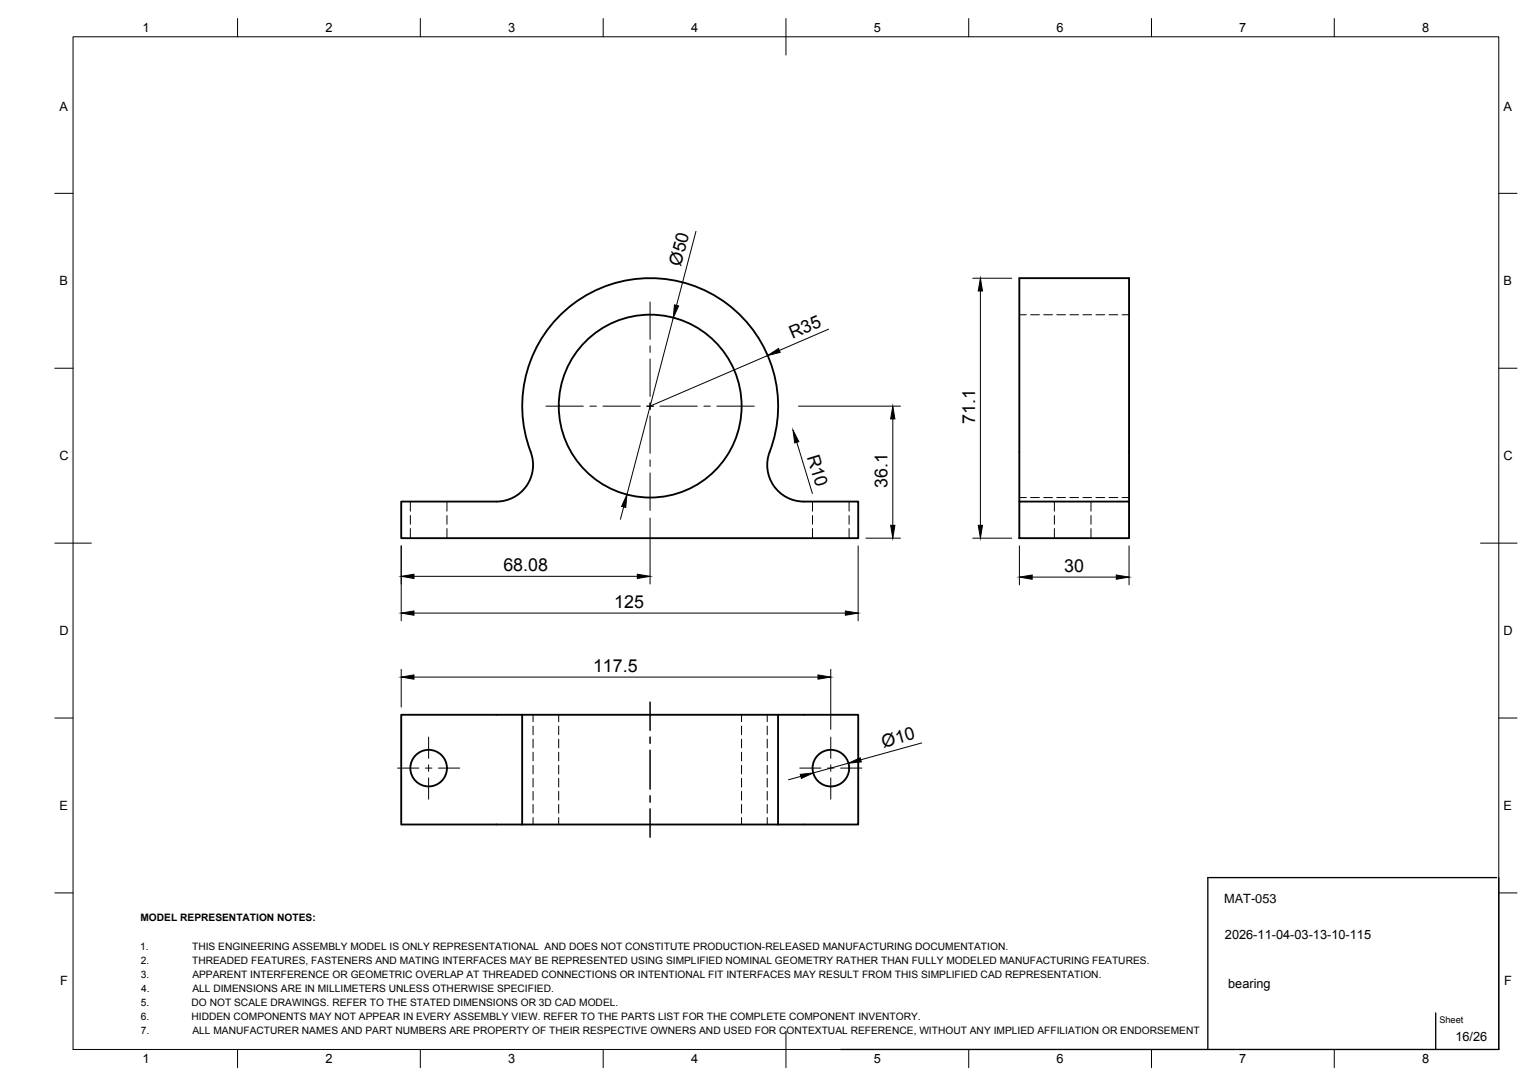
ISO-10303-21;
HEADER;
FILE_DESCRIPTION (('STEP AP214'),
    '1' );
FILE_NAME ('bearing.step',
    '2026-10-10T03:43:58',
    ( '' ),
    ( '' ),
    'SwSTEP 2.0',
    'SolidWorks 2026',
    '' );
FILE_SCHEMA (( 'AUTOMOTIVE_DESIGN' ));
ENDSEC;

DATA;
#80=( NAMED_UNIT ( * ) PLANE_ANGLE_UNIT ( ) SI_UNIT ( $, .RADIAN. ) );
#94=EDGE_CURVE ( 'NONE', #10885, #49715, #23914, .T. ) ;
#206=EDGE_CURVE ( 'NONE', #68800, #69210, #4699, .T. ) ;
#264=( NAMED_UNIT ( * ) SI_UNIT ( $, .STERADIAN. ) SOLID_ANGLE_UNIT ( ) );
#321=EDGE_CURVE ( 'NONE', #69231, #19186, #17084, .T. ) ;
#468=DIRECTION ( 'NONE',  ( -0.000000000000000000, -0.000000000000000000, -1.000000000000000000 ) ) ;
#638=ORIENTED_EDGE ( 'NONE', *, *, #35254, .T. ) ;
#689=ORIENTED_EDGE ( 'NONE', *, *, #206, .F. ) ;
#727=DIRECTION ( 'NONE',  ( -0.000000000000000000, -0.000000000000000000, -1.000000000000000000 ) ) ;
#740=CARTESIAN_POINT ( 'NONE',  ( -56.92000000000000171, -36.09918303830819752, 30.00000000000000000 ) ) ;
#794=LINE ( 'NONE', #10991, #2437 ) ;
#842=ORIENTED_EDGE ( 'NONE', *, *, #61547, .F. ) ;
#853=ORIENTED_EDGE ( 'NONE', *, *, #16095, .T. ) ;
#901=EDGE_CURVE ( 'NONE', #59026, #60171, #23772, .T. ) ;
#1272=CARTESIAN_POINT ( 'NONE',  ( 60.58000000000000540, -36.09918303830819752, 15.41169613715280562 ) ) ;
#1543=CARTESIAN_POINT ( 'NONE',  ( 0.000000000000000000, -26.09918303830819397, 0.000000000000000000 ) ) ;
#1613=VECTOR ( 'NONE', #727, 1000.000000000000000 ) ;
#1651=DIRECTION ( 'NONE',  ( 1.000000000000000000, 0.000000000000000000, 0.000000000000000000 ) ) ;
#2060=VERTEX_POINT ( 'NONE', #27925 ) ;
#2101=EDGE_CURVE ( 'NONE', #34582, #25022, #49713, .T. ) ;
#2170=FACE_BOUND ( 'NONE', #11561, .T. ) ;
#2203=DIRECTION ( 'NONE',  ( 0.000000000000000000, -0.000000000000000000, 1.000000000000000000 ) ) ;
#2389=ADVANCED_FACE ( 'NONE', ( #2170, #50353, #34538 ), #24324, .F. ) ;
#2437=VECTOR ( 'NONE', #32455, 1000.000000000000000 ) ;
#2467=ORIENTED_EDGE ( 'NONE', *, *, #66746, .T. ) ;
#2987=ORIENTED_EDGE ( 'NONE', *, *, #39684, .T. ) ;
#3166=CARTESIAN_POINT ( 'NONE',  ( 0.000000000000000000, 0.000000000000000000, 0.000000000000000000 ) ) ;
#3233=DIRECTION ( 'NONE',  ( -0.000000000000000000, 0.000000000000000000, 1.000000000000000000 ) ) ;
#3268=FACE_OUTER_BOUND ( 'NONE', #19540, .T. ) ;
#3274=LINE ( 'NONE', #47533, #24176 ) ;
#3390=EDGE_LOOP ( 'NONE', ( #67378, #26917 ) ) ;
#3419=ORIENTED_EDGE ( 'NONE', *, *, #42188, .T. ) ;
#3531=DIRECTION ( 'NONE',  ( 0.000000000000000000, 0.000000000000000000, 1.000000000000000000 ) ) ;
#3669=DIRECTION ( 'NONE',  ( -1.000000000000000000, 0.000000000000000000, 0.000000000000000000 ) ) ;
#3748=ORIENTED_EDGE ( 'NONE', *, *, #63637, .F. ) ;
#3791=AXIS2_PLACEMENT_3D ( 'NONE', #56338, #3233, #51757 ) ;
#4023=PLANE ( 'NONE',  #21900 ) ;
#4189=CIRCLE ( 'NONE', #54729, 9.999999999999994671 ) ;
#4235=CIRCLE ( 'NONE', #8711, 35.00000000000000000 ) ;
#4337=UNCERTAINTY_MEASURE_WITH_UNIT (LENGTH_MEASURE( 1.000000000000000082E-05 ), #21203, 'distance_accuracy_value', 'NONE');
#4385=ORIENTED_EDGE ( 'NONE', *, *, #37619, .F. ) ;
#4422=CIRCLE ( 'NONE', #29131, 35.00000000000000000 ) ;
#4581=DIRECTION ( 'NONE',  ( 0.000000000000000000, -1.000000000000000000, 0.000000000000000000 ) ) ;
#4699=CIRCLE ( 'NONE', #30626, 25.00000000000000000 ) ;
#4744=AXIS2_PLACEMENT_3D ( 'NONE', #11177, #37921, #48791 ) ;
#4759=DIRECTION ( 'NONE',  ( -1.000000000000000000, 0.000000000000000000, 0.000000000000000000 ) ) ;
#4795=CARTESIAN_POINT ( 'NONE',  ( 42.02161712141799654, -16.09918303830818687, 30.00000000000000000 ) ) ;
#4926=AXIS2_PLACEMENT_3D ( 'NONE', #54248, #48974, #54958 ) ;
#4990=AXIS2_PLACEMENT_3D ( 'NONE', #28858, #13370, #13032 ) ;
#5047=CARTESIAN_POINT ( 'NONE',  ( 32.68347998332510684, -12.52158680757303344, 0.000000000000000000 ) ) ;
#5120=ORIENTED_EDGE ( 'NONE', *, *, #47618, .T. ) ;
#5137=ADVANCED_FACE ( 'NONE', ( #56258 ), #41479, .F. ) ;
#5265=CARTESIAN_POINT ( 'NONE',  ( -32.68347998332510684, -12.52158680757305298, 30.00000000000000000 ) ) ;
#5279=DIRECTION ( 'NONE',  ( -0.000000000000000000, 0.000000000000000000, 1.000000000000000000 ) ) ;
#5478=FACE_OUTER_BOUND ( 'NONE', #49318, .T. ) ;
#5519=AXIS2_PLACEMENT_3D ( 'NONE', #49067, #10758, #32225 ) ;
#5525=CARTESIAN_POINT ( 'NONE',  ( -32.68347998332510684, -12.52158680757305298, 30.00000000000000000 ) ) ;
#5684=EDGE_LOOP ( 'NONE', ( #29474, #21632, #30647, #66868, #13949, #638, #26967, #48733, #66037, #63383, #37601 ) ) ;
#5699=SHAPE_REPRESENTATION_RELATIONSHIP ( 'NONE' , 'NONE' ,  #52783, #13951 ) ;
#5790=ORIENTED_EDGE ( 'NONE', *, *, #62827, .F. ) ;
#5793=VECTOR ( 'NONE', #13746, 1000.000000000000000 ) ;
#5839=DIRECTION ( 'NONE',  ( 0.000000000000000000, 0.000000000000000000, 1.000000000000000000 ) ) ;
#5937=EDGE_CURVE ( 'NONE', #68965, #62166, #22348, .T. ) ;
#5949=LINE ( 'NONE', #17200, #47356 ) ;
#6014=ORIENTED_EDGE ( 'NONE', *, *, #39684, .F. ) ;
#6019=EDGE_CURVE ( 'NONE', #54796, #68965, #27476, .T. ) ;
#6266=CYLINDRICAL_SURFACE ( 'NONE', #25796, 25.00000000000000000 ) ;
#6343=EDGE_LOOP ( 'NONE', ( #7440, #64244, #49324, #19712 ) ) ;
#6359=ADVANCED_FACE ( 'NONE', ( #33781 ), #61552, .F. ) ;
#6804=ADVANCED_FACE ( 'NONE', ( #52968 ), #26260, .F. ) ;
#7182=UNCERTAINTY_MEASURE_WITH_UNIT (LENGTH_MEASURE( 1.000000000000000082E-05 ), #26664, 'distance_accuracy_value', 'NONE');
#7284=CARTESIAN_POINT ( 'NONE',  ( 0.000000000000000000, -26.09918303830819397, 0.000000000000000000 ) ) ;
#7326=VERTEX_POINT ( 'NONE', #740 ) ;
#7385=ADVANCED_FACE ( 'NONE', ( #13051, #33099 ), #22539, .T. ) ;
#7440=ORIENTED_EDGE ( 'NONE', *, *, #69569, .F. ) ;
#7470=EDGE_CURVE ( 'NONE', #64129, #56353, #61901, .T. ) ;
#7778=ORIENTED_EDGE ( 'NONE', *, *, #45908, .F. ) ;
#7912=ORIENTED_EDGE ( 'NONE', *, *, #206, .T. ) ;
#8044=DIRECTION ( 'NONE',  ( -0.000000000000000000, -0.000000000000000000, -1.000000000000000000 ) ) ;
#8085=EDGE_LOOP ( 'NONE', ( #35440, #41087, #18841, #5790 ) ) ;
#8134=CARTESIAN_POINT ( 'NONE',  ( 0.000000000000000000, -36.09918303830819752, 30.00000000000000000 ) ) ;
#8162=CARTESIAN_POINT ( 'NONE',  ( 60.58000000000000540, -26.09918303830819397, 10.41169613715280740 ) ) ;
#8209=AXIS2_PLACEMENT_3D ( 'NONE', #61244, #56654, #3531 ) ;
#8319=DIRECTION ( 'NONE',  ( 1.000000000000000000, 0.000000000000000000, 0.000000000000000000 ) ) ;
#8388=VERTEX_POINT ( 'NONE', #32337 ) ;
#8554=EDGE_LOOP ( 'NONE', ( #37579, #50255 ) ) ;
#8596=ORIENTED_EDGE ( 'NONE', *, *, #16636, .T. ) ;
#8711=AXIS2_PLACEMENT_3D ( 'NONE', #20766, #5279, #53448 ) ;
#8727=DIRECTION ( 'NONE',  ( 1.000000000000000000, 0.000000000000000000, 0.000000000000000000 ) ) ;
#8957=FACE_OUTER_BOUND ( 'NONE', #20268, .T. ) ;
#9217=VECTOR ( 'NONE', #1651, 1000.000000000000000 ) ;
#9390=APPLICATION_CONTEXT ( 'automotive_design' ) ;
#9517=EDGE_LOOP ( 'NONE', ( #61861, #65426, #23642, #69064 ) ) ;
#9565=ADVANCED_FACE ( 'NONE', ( #10850 ), #27364, .F. ) ;
#10006=( GEOMETRIC_REPRESENTATION_CONTEXT ( 3 ) GLOBAL_UNCERTAINTY_ASSIGNED_CONTEXT ( ( #7182 ) ) GLOBAL_UNIT_ASSIGNED_CONTEXT ( ( #26664, #21379, #264 ) ) REPRESENTATION_CONTEXT ( 'NONE', 'WORKASPACE' ) );
#10336=DIRECTION ( 'NONE',  ( -0.000000000000000000, 0.000000000000000000, 1.000000000000000000 ) ) ;
#10758=DIRECTION ( 'NONE',  ( -0.000000000000000000, -0.000000000000000000, -1.000000000000000000 ) ) ;
#10850=FACE_OUTER_BOUND ( 'NONE', #63710, .T. ) ;
#10885=VERTEX_POINT ( 'NONE', #46687 ) ;
#10991=CARTESIAN_POINT ( 'NONE',  ( 0.000000000000000000, -26.09918303830819397, 30.00000000000000000 ) ) ;
#11023=VERTEX_POINT ( 'NONE', #59646 ) ;
#11066=CARTESIAN_POINT ( 'NONE',  ( -49.42000000000000171, -26.09918303830819397, 20.41169613715280207 ) ) ;
#11177=CARTESIAN_POINT ( 'NONE',  ( 60.58000000000000540, -26.09918303830819397, 15.41169613715280562 ) ) ;
#11201=CYLINDRICAL_SURFACE ( 'NONE', #29050, 35.00000000000000000 ) ;
#11314=CIRCLE ( 'NONE', #55152, 4.999999999999997335 ) ;
#11561=EDGE_LOOP ( 'NONE', ( #41589, #853 ) ) ;
#11646=LINE ( 'NONE', #27836, #12727 ) ;
#11924=EDGE_CURVE ( 'NONE', #69210, #11023, #67920, .T. ) ;
#12007=ORIENTED_EDGE ( 'NONE', *, *, #15952, .F. ) ;
#12261=COLOUR_RGB ( '',0.7921568627450980005, 0.8196078431372548767, 0.9333333333333333481 ) ;
#12270=ORIENTED_EDGE ( 'NONE', *, *, #30171, .T. ) ;
#12727=VECTOR ( 'NONE', #39433, 1000.000000000000000 ) ;
#13032=DIRECTION ( 'NONE',  ( 0.000000000000000000, 0.000000000000000000, 1.000000000000000000 ) ) ;
#13051=FACE_BOUND ( 'NONE', #60200, .T. ) ;
#13366=CARTESIAN_POINT ( 'NONE',  ( 68.07999999999999829, -36.09918303830819752, 30.00000000000000000 ) ) ;
#13370=DIRECTION ( 'NONE',  ( -0.000000000000000000, 1.000000000000000000, -0.000000000000000000 ) ) ;
#13541=CIRCLE ( 'NONE', #40490, 9.999999999999994671 ) ;
#13645=CARTESIAN_POINT ( 'NONE',  ( -56.92000000000000171, -26.09918303830819397, 30.00000000000000000 ) ) ;
#13746=DIRECTION ( 'NONE',  ( 1.000000000000000000, 0.000000000000000000, 0.000000000000000000 ) ) ;
#13949=ORIENTED_EDGE ( 'NONE', *, *, #32634, .F. ) ;
#13951=ADVANCED_BREP_SHAPE_REPRESENTATION ( '', ( #64527, #66832 ), #47807 ) ;
#14404=CARTESIAN_POINT ( 'NONE',  ( -49.42000000000000171, -36.09918303830819752, 15.41169613715280562 ) ) ;
#14569=VECTOR ( 'NONE', #468, 1000.000000000000000 ) ;
#14703=ORIENTED_EDGE ( 'NONE', *, *, #39776, .T. ) ;
#14738=ORIENTED_EDGE ( 'NONE', *, *, #18028, .F. ) ;
#14973=DIRECTION ( 'NONE',  ( -0.000000000000000000, 0.000000000000000000, 1.000000000000000000 ) ) ;
#15094=AXIS2_PLACEMENT_3D ( 'NONE', #56100, #30402, #67361 ) ;
#15197=FACE_BOUND ( 'NONE', #25741, .T. ) ;
#15203=DIRECTION ( 'NONE',  ( -0.000000000000000000, -0.000000000000000000, -1.000000000000000000 ) ) ;
#15268=PRODUCT_DEFINITION_SHAPE ( 'NONE', 'NONE',  #16010 ) ;
#15306=ORIENTED_EDGE ( 'NONE', *, *, #62917, .T. ) ;
#15422=FILL_AREA_STYLE_COLOUR ( '', #12261 ) ;
#15428=CARTESIAN_POINT ( 'NONE',  ( -42.02161712141799654, -26.09918303830819042, 30.00000000000000000 ) ) ;
#15522=AXIS2_PLACEMENT_3D ( 'NONE', #19120, #61686, #65951 ) ;
#15524=ORIENTED_EDGE ( 'NONE', *, *, #17794, .T. ) ;
#15762=SURFACE_STYLE_USAGE ( .BOTH. , #27000 ) ;
#15841=LINE ( 'NONE', #22159, #59706 ) ;
#15915=CARTESIAN_POINT ( 'NONE',  ( 60.58000000000000540, -36.09918303830819752, 15.41169613715280562 ) ) ;
#15952=EDGE_CURVE ( 'NONE', #69210, #68800, #27088, .T. ) ;
#16010=PRODUCT_DEFINITION ( 'UNKNOWN', '', #38892, #48581 ) ;
#16095=EDGE_CURVE ( 'NONE', #51430, #38471, #11314, .T. ) ;
#16106=ORIENTED_EDGE ( 'NONE', *, *, #2101, .F. ) ;
#16225=VECTOR ( 'NONE', #55096, 1000.000000000000000 ) ;
#16364=CARTESIAN_POINT ( 'NONE',  ( -56.92000000000000171, -26.09918303830819397, 0.000000000000000000 ) ) ;
#16415=ORIENTED_EDGE ( 'NONE', *, *, #42188, .F. ) ;
#16636=EDGE_CURVE ( 'NONE', #18961, #49715, #39787, .T. ) ;
#17084=CIRCLE ( 'NONE', #4744, 4.999999999999997335 ) ;
#17200=CARTESIAN_POINT ( 'NONE',  ( -56.92000000000000171, 0.000000000000000000, 0.000000000000000000 ) ) ;
#17253=DIRECTION ( 'NONE',  ( 0.000000000000000000, 1.000000000000000000, 0.000000000000000000 ) ) ;
#17301=DIRECTION ( 'NONE',  ( 0.000000000000000000, 1.000000000000000000, -0.000000000000000000 ) ) ;
#17421=ORIENTED_EDGE ( 'NONE', *, *, #7470, .F. ) ;
#17493=ORIENTED_EDGE ( 'NONE', *, *, #22963, .F. ) ;
#17694=VECTOR ( 'NONE', #63460, 1000.000000000000000 ) ;
#17709=ORIENTED_EDGE ( 'NONE', *, *, #35255, .T. ) ;
#17794=EDGE_CURVE ( 'NONE', #64838, #18961, #5949, .T. ) ;
#17887=CARTESIAN_POINT ( 'NONE',  ( -49.42000000000000171, -36.09918303830819752, 10.41169613715280740 ) ) ;
#17943=EDGE_CURVE ( 'NONE', #64838, #47377, #60396, .T. ) ;
#18028=EDGE_CURVE ( 'NONE', #2060, #60359, #15841, .T. ) ;
#18201=CARTESIAN_POINT ( 'NONE',  ( 60.58000000000000540, -36.09918303830819752, 20.41169613715280207 ) ) ;
#18308=ORIENTED_EDGE ( 'NONE', *, *, #61547, .T. ) ;
#18372=ORIENTED_EDGE ( 'NONE', *, *, #69569, .T. ) ;
#18841=ORIENTED_EDGE ( 'NONE', *, *, #35254, .F. ) ;
#18961=VERTEX_POINT ( 'NONE', #26497 ) ;
#19067=EDGE_CURVE ( 'NONE', #55170, #60171, #59649, .T. ) ;
#19120=CARTESIAN_POINT ( 'NONE',  ( 0.000000000000000000, 0.000000000000000000, 0.000000000000000000 ) ) ;
#19186=VERTEX_POINT ( 'NONE', #8162 ) ;
#19322=ADVANCED_FACE ( 'NONE', ( #52624 ), #57571, .F. ) ;
#19540=EDGE_LOOP ( 'NONE', ( #63713, #12270, #61069, #48577, #4385, #63890, #50946, #25404, #56667, #38404, #17709 ) ) ;
#19562=DIRECTION ( 'NONE',  ( -0.000000000000000000, -0.000000000000000000, -1.000000000000000000 ) ) ;
#19583=DIRECTION ( 'NONE',  ( -0.000000000000000000, -0.000000000000000000, -1.000000000000000000 ) ) ;
#19712=ORIENTED_EDGE ( 'NONE', *, *, #32634, .T. ) ;
#19717=DIRECTION ( 'NONE',  ( -0.000000000000000000, -0.000000000000000000, -1.000000000000000000 ) ) ;
#19921=PRODUCT_CONTEXT ( 'NONE', #68260, 'mechanical' ) ;
#20033=FACE_BOUND ( 'NONE', #58971, .T. ) ;
#20268=EDGE_LOOP ( 'NONE', ( #7912, #29670, #42435, #16415 ) ) ;
#20692=AXIS2_PLACEMENT_3D ( 'NONE', #44864, #67038, #24464 ) ;
#20766=CARTESIAN_POINT ( 'NONE',  ( 0.000000000000000000, 0.000000000000000000, 30.00000000000000000 ) ) ;
#20798=AXIS2_PLACEMENT_3D ( 'NONE', #51587, #14973, #24853 ) ;
#20804=CARTESIAN_POINT ( 'NONE',  ( -42.02161712141799654, -26.09918303830819042, 30.00000000000000000 ) ) ;
#20846=DIRECTION ( 'NONE',  ( 0.000000000000000000, 0.000000000000000000, 1.000000000000000000 ) ) ;
#20961=CARTESIAN_POINT ( 'NONE',  ( 60.58000000000000540, -36.09918303830819752, 15.41169613715280562 ) ) ;
#20997=AXIS2_PLACEMENT_3D ( 'NONE', #63509, #19562, #4759 ) ;
#21026=CARTESIAN_POINT ( 'NONE',  ( 42.02161712141799654, -16.09918303830818687, 30.00000000000000000 ) ) ;
#21055=CIRCLE ( 'NONE', #22145, 4.999999999999997335 ) ;
#21159=DIRECTION ( 'NONE',  ( -0.000000000000000000, -0.000000000000000000, -1.000000000000000000 ) ) ;
#21203=( LENGTH_UNIT ( ) NAMED_UNIT ( * ) SI_UNIT ( .MILLI., .METRE. ) );
#21379=( NAMED_UNIT ( * ) PLANE_ANGLE_UNIT ( ) SI_UNIT ( $, .RADIAN. ) );
#21493=AXIS2_PLACEMENT_3D ( 'NONE', #41734, #19583, #62145 ) ;
#21632=ORIENTED_EDGE ( 'NONE', *, *, #62427, .F. ) ;
#21900=AXIS2_PLACEMENT_3D ( 'NONE', #64135, #57834, #37063 ) ;
#22145=AXIS2_PLACEMENT_3D ( 'NONE', #15915, #31746, #20846 ) ;
#22159=CARTESIAN_POINT ( 'NONE',  ( -49.42000000000000171, -36.09918303830819752, 20.41169613715280207 ) ) ;
#22203=CARTESIAN_POINT ( 'NONE',  ( 0.000000000000000000, 0.000000000000000000, 30.00000000000000000 ) ) ;
#22348=LINE ( 'NONE', #38171, #40951 ) ;
#22414=DIRECTION ( 'NONE',  ( 0.000000000000000000, 0.000000000000000000, 1.000000000000000000 ) ) ;
#22539=PLANE ( 'NONE',  #61287 ) ;
#22576=CARTESIAN_POINT ( 'NONE',  ( 42.02161712141799654, -26.09918303830819042, 30.00000000000000000 ) ) ;
#22731=EDGE_CURVE ( 'NONE', #8388, #25022, #64796, .T. ) ;
#22765=ORIENTED_EDGE ( 'NONE', *, *, #24864, .T. ) ;
#22917=VECTOR ( 'NONE', #37027, 1000.000000000000000 ) ;
#22963=EDGE_CURVE ( 'NONE', #25022, #49715, #45777, .T. ) ;
#23028=AXIS2_PLACEMENT_3D ( 'NONE', #52625, #25911, #47338 ) ;
#23059=VECTOR ( 'NONE', #31223, 1000.000000000000000 ) ;
#23230=AXIS2_PLACEMENT_3D ( 'NONE', #58157, #59518, #53201 ) ;
#23241=LINE ( 'NONE', #38005, #1613 ) ;
#23549=FACE_OUTER_BOUND ( 'NONE', #31909, .T. ) ;
#23630=CARTESIAN_POINT ( 'NONE',  ( -42.02161712141799654, -26.09918303830819042, 0.000000000000000000 ) ) ;
#23642=ORIENTED_EDGE ( 'NONE', *, *, #43707, .T. ) ;
#23686=VECTOR ( 'NONE', #61208, 1000.000000000000000 ) ;
#23772=LINE ( 'NONE', #33981, #47468 ) ;
#23802=CARTESIAN_POINT ( 'NONE',  ( 35.00000000000000000, 4.286263797015736496E-15, 30.00000000000000000 ) ) ;
#23912=DIRECTION ( 'NONE',  ( 0.000000000000000000, 0.000000000000000000, 1.000000000000000000 ) ) ;
#23914=LINE ( 'NONE', #13366, #50749 ) ;
#23916=ORIENTED_EDGE ( 'NONE', *, *, #17943, .F. ) ;
#24016=DIRECTION ( 'NONE',  ( -0.000000000000000000, 0.000000000000000000, 1.000000000000000000 ) ) ;
#24032=CARTESIAN_POINT ( 'NONE',  ( 42.02161712141799654, -26.09918303830819042, 0.000000000000000000 ) ) ;
#24176=VECTOR ( 'NONE', #15203, 1000.000000000000000 ) ;
#24280=LINE ( 'NONE', #61890, #23686 ) ;
#24324=PLANE ( 'NONE',  #57730 ) ;
#24378=ORIENTED_EDGE ( 'NONE', *, *, #24864, .F. ) ;
#24464=DIRECTION ( 'NONE',  ( 1.000000000000000000, 0.000000000000000000, 0.000000000000000000 ) ) ;
#24624=AXIS2_PLACEMENT_3D ( 'NONE', #24791, #30071, #3669 ) ;
#24791=CARTESIAN_POINT ( 'NONE',  ( 0.000000000000000000, 0.000000000000000000, 30.00000000000000000 ) ) ;
#24853=DIRECTION ( 'NONE',  ( 1.000000000000000000, 0.000000000000000000, 0.000000000000000000 ) ) ;
#24864=EDGE_CURVE ( 'NONE', #11023, #40688, #28695, .T. ) ;
#24930=CYLINDRICAL_SURFACE ( 'NONE', #26617, 35.00000000000000000 ) ;
#25022=VERTEX_POINT ( 'NONE', #61011 ) ;
#25318=FACE_OUTER_BOUND ( 'NONE', #5684, .T. ) ;
#25404=ORIENTED_EDGE ( 'NONE', *, *, #30518, .T. ) ;
#25516=ORIENTED_EDGE ( 'NONE', *, *, #901, .F. ) ;
#25549=FACE_OUTER_BOUND ( 'NONE', #6343, .T. ) ;
#25741=EDGE_LOOP ( 'NONE', ( #689, #12007 ) ) ;
#25796=AXIS2_PLACEMENT_3D ( 'NONE', #38277, #65373, #44606 ) ;
#25837=LINE ( 'NONE', #47951, #17694 ) ;
#25902=DIRECTION ( 'NONE',  ( 0.000000000000000000, 0.000000000000000000, 1.000000000000000000 ) ) ;
#25911=DIRECTION ( 'NONE',  ( 1.000000000000000000, 0.000000000000000000, -0.000000000000000000 ) ) ;
#26184=AXIS2_PLACEMENT_3D ( 'NONE', #54403, #54757, #22414 ) ;
#26260=CYLINDRICAL_SURFACE ( 'NONE', #57872, 10.00000000000000178 ) ;
#26469=ORIENTED_EDGE ( 'NONE', *, *, #53883, .T. ) ;
#26497=CARTESIAN_POINT ( 'NONE',  ( -56.92000000000000171, -36.09918303830819752, 0.000000000000000000 ) ) ;
#26617=AXIS2_PLACEMENT_3D ( 'NONE', #50273, #29165, #29855 ) ;
#26644=ORIENTED_EDGE ( 'NONE', *, *, #19067, .T. ) ;
#26664=( LENGTH_UNIT ( ) NAMED_UNIT ( * ) SI_UNIT ( .MILLI., .METRE. ) );
#26697=ORIENTED_EDGE ( 'NONE', *, *, #54212, .F. ) ;
#26917=ORIENTED_EDGE ( 'NONE', *, *, #39776, .F. ) ;
#26936=FACE_OUTER_BOUND ( 'NONE', #36952, .T. ) ;
#26967=ORIENTED_EDGE ( 'NONE', *, *, #55000, .T. ) ;
#26980=DIRECTION ( 'NONE',  ( -0.000000000000000000, 0.000000000000000000, 1.000000000000000000 ) ) ;
#27000=SURFACE_SIDE_STYLE ('',( #31946 ) ) ;
#27088=CIRCLE ( 'NONE', #28195, 25.00000000000000000 ) ;
#27157=DIRECTION ( 'NONE',  ( 0.000000000000000000, 0.000000000000000000, 1.000000000000000000 ) ) ;
#27276=DIRECTION ( 'NONE',  ( -1.000000000000000000, 0.000000000000000000, 0.000000000000000000 ) ) ;
#27355=CIRCLE ( 'NONE', #4926, 4.999999999999997335 ) ;
#27364=CYLINDRICAL_SURFACE ( 'NONE', #33371, 4.999999999999997335 ) ;
#27476=CIRCLE ( 'NONE', #15094, 10.00000000000000178 ) ;
#27578=VECTOR ( 'NONE', #57333, 1000.000000000000000 ) ;
#27634=VERTEX_POINT ( 'NONE', #60545 ) ;
#27731=FACE_OUTER_BOUND ( 'NONE', #30142, .T. ) ;
#27836=CARTESIAN_POINT ( 'NONE',  ( 60.58000000000000540, -36.09918303830819752, 20.41169613715280207 ) ) ;
#27925=CARTESIAN_POINT ( 'NONE',  ( -49.42000000000000171, -36.09918303830819752, 20.41169613715280207 ) ) ;
#28081=CARTESIAN_POINT ( 'NONE',  ( -42.02161712141799654, -16.09918303830819397, 30.00000000000000000 ) ) ;
#28152=CARTESIAN_POINT ( 'NONE',  ( 60.58000000000000540, -36.09918303830819752, 10.41169613715280740 ) ) ;
#28195=AXIS2_PLACEMENT_3D ( 'NONE', #35448, #49970, #8727 ) ;
#28411=ORIENTED_EDGE ( 'NONE', *, *, #43876, .T. ) ;
#28532=CARTESIAN_POINT ( 'NONE',  ( 0.000000000000000000, -26.09918303830819397, 30.00000000000000000 ) ) ;
#28695=CIRCLE ( 'NONE', #20798, 25.00000000000000000 ) ;
#28818=ORIENTED_EDGE ( 'NONE', *, *, #94, .F. ) ;
#28858=CARTESIAN_POINT ( 'NONE',  ( -49.42000000000000171, -36.09918303830819752, 15.41169613715280562 ) ) ;
#28938=CARTESIAN_POINT ( 'NONE',  ( 0.000000000000000000, -26.09918303830819397, 30.00000000000000000 ) ) ;
#28955=CARTESIAN_POINT ( 'NONE',  ( 0.000000000000000000, 0.000000000000000000, 0.000000000000000000 ) ) ;
#29050=AXIS2_PLACEMENT_3D ( 'NONE', #38287, #37244, #37942 ) ;
#29131=AXIS2_PLACEMENT_3D ( 'NONE', #35336, #39572, #50472 ) ;
#29165=DIRECTION ( 'NONE',  ( -0.000000000000000000, -0.000000000000000000, -1.000000000000000000 ) ) ;
#29285=ORIENTED_EDGE ( 'NONE', *, *, #35255, .F. ) ;
#29474=ORIENTED_EDGE ( 'NONE', *, *, #17943, .T. ) ;
#29477=DIRECTION ( 'NONE',  ( -0.000000000000000000, -0.000000000000000000, -1.000000000000000000 ) ) ;
#29556=ADVANCED_FACE ( 'NONE', ( #25549 ), #37116, .T. ) ;
#29620=ADVANCED_FACE ( 'NONE', ( #23549 ), #24930, .T. ) ;
#29670=ORIENTED_EDGE ( 'NONE', *, *, #11924, .T. ) ;
#29855=DIRECTION ( 'NONE',  ( -1.000000000000000000, 0.000000000000000000, 0.000000000000000000 ) ) ;
#30071=DIRECTION ( 'NONE',  ( -0.000000000000000000, -0.000000000000000000, -1.000000000000000000 ) ) ;
#30142=EDGE_LOOP ( 'NONE', ( #65328, #18372, #26644, #25516 ) ) ;
#30171=EDGE_CURVE ( 'NONE', #42155, #7326, #68016, .T. ) ;
#30254=EDGE_CURVE ( 'NONE', #38471, #51430, #21055, .T. ) ;
#30402=DIRECTION ( 'NONE',  ( -0.000000000000000000, 0.000000000000000000, 1.000000000000000000 ) ) ;
#30518=EDGE_CURVE ( 'NONE', #54796, #27634, #4235, .T. ) ;
#30626=AXIS2_PLACEMENT_3D ( 'NONE', #30931, #36202, #52373 ) ;
#30647=ORIENTED_EDGE ( 'NONE', *, *, #62917, .F. ) ;
#30833=FACE_OUTER_BOUND ( 'NONE', #59558, .T. ) ;
#30843=CARTESIAN_POINT ( 'NONE',  ( -49.42000000000000171, -26.09918303830819397, 10.41169613715280740 ) ) ;
#30931=CARTESIAN_POINT ( 'NONE',  ( 0.000000000000000000, 0.000000000000000000, 30.00000000000000000 ) ) ;
#31015=EDGE_LOOP ( 'NONE', ( #23916, #7778, #28411, #43766 ) ) ;
#31193=PLANE ( 'NONE',  #23028 ) ;
#31223=DIRECTION ( 'NONE',  ( 1.000000000000000000, 0.000000000000000000, 0.000000000000000000 ) ) ;
#31746=DIRECTION ( 'NONE',  ( 0.000000000000000000, 1.000000000000000000, -0.000000000000000000 ) ) ;
#31909=EDGE_LOOP ( 'NONE', ( #3748, #69400, #15306, #39862 ) ) ;
#31946=SURFACE_STYLE_FILL_AREA ( #36882 ) ;
#32148=DIRECTION ( 'NONE',  ( 1.000000000000000000, 0.000000000000000000, 0.000000000000000000 ) ) ;
#32160=EDGE_LOOP ( 'NONE', ( #16106, #59838, #33744, #49558 ) ) ;
#32224=EDGE_CURVE ( 'NONE', #7326, #10885, #64206, .T. ) ;
#32225=DIRECTION ( 'NONE',  ( -1.000000000000000000, 0.000000000000000000, 0.000000000000000000 ) ) ;
#32235=ADVANCED_FACE ( 'NONE', ( #30833 ), #36450, .F. ) ;
#32319=DIRECTION ( 'NONE',  ( -0.000000000000000000, 1.000000000000000000, -0.000000000000000000 ) ) ;
#32337=CARTESIAN_POINT ( 'NONE',  ( 68.07999999999999829, -26.09918303830819397, 30.00000000000000000 ) ) ;
#32455=DIRECTION ( 'NONE',  ( 1.000000000000000000, 0.000000000000000000, 0.000000000000000000 ) ) ;
#32634=EDGE_CURVE ( 'NONE', #56777, #55170, #4422, .T. ) ;
#32991=CARTESIAN_POINT ( 'NONE',  ( -42.02161712141799654, -16.09918303830819397, 0.000000000000000000 ) ) ;
#33003=CARTESIAN_POINT ( 'NONE',  ( 60.58000000000000540, -36.09918303830819752, 15.41169613715280562 ) ) ;
#33018=CARTESIAN_POINT ( 'NONE',  ( 42.02161712141799654, -16.09918303830818687, 0.000000000000000000 ) ) ;
#33099=FACE_OUTER_BOUND ( 'NONE', #31015, .T. ) ;
#33207=ADVANCED_FACE ( 'NONE', ( #26936 ), #54702, .F. ) ;
#33357=DIRECTION ( 'NONE',  ( 1.000000000000000000, 0.000000000000000000, 0.000000000000000000 ) ) ;
#33371=AXIS2_PLACEMENT_3D ( 'NONE', #33003, #32319, #65725 ) ;
#33467=AXIS2_PLACEMENT_3D ( 'NONE', #28955, #24016, #66254 ) ;
#33555=EDGE_CURVE ( 'NONE', #7326, #18961, #58507, .T. ) ;
#33744=ORIENTED_EDGE ( 'NONE', *, *, #37619, .T. ) ;
#33781=FACE_OUTER_BOUND ( 'NONE', #44217, .T. ) ;
#33811=LINE ( 'NONE', #28532, #23059 ) ;
#33919=EDGE_CURVE ( 'NONE', #49926, #47377, #69336, .T. ) ;
#33981=CARTESIAN_POINT ( 'NONE',  ( -35.00000000000000000, 0.000000000000000000, 30.00000000000000000 ) ) ;
#34018=AXIS2_PLACEMENT_3D ( 'NONE', #28938, #66238, #2203 ) ;
#34294=ADVANCED_FACE ( 'NONE', ( #59722 ), #6266, .F. ) ;
#34538=FACE_OUTER_BOUND ( 'NONE', #52695, .T. ) ;
#34582=VERTEX_POINT ( 'NONE', #24032 ) ;
#34585=CIRCLE ( 'NONE', #33467, 35.00000000000000000 ) ;
#35254=EDGE_CURVE ( 'NONE', #56777, #62166, #66334, .T. ) ;
#35255=EDGE_CURVE ( 'NONE', #69403, #49926, #13541, .T. ) ;
#35336=CARTESIAN_POINT ( 'NONE',  ( 0.000000000000000000, 0.000000000000000000, 0.000000000000000000 ) ) ;
#35440=ORIENTED_EDGE ( 'NONE', *, *, #6019, .T. ) ;
#35448=CARTESIAN_POINT ( 'NONE',  ( 0.000000000000000000, 0.000000000000000000, 30.00000000000000000 ) ) ;
#35554=CARTESIAN_POINT ( 'NONE',  ( 25.00000000000000000, 3.061616997868383043E-15, 30.00000000000000000 ) ) ;
#35692=CARTESIAN_POINT ( 'NONE',  ( 32.02161712141799654, -16.09918303830818687, 0.000000000000000000 ) ) ;
#35999=CARTESIAN_POINT ( 'NONE',  ( -56.92000000000000171, 0.000000000000000000, 30.00000000000000000 ) ) ;
#36202=DIRECTION ( 'NONE',  ( -0.000000000000000000, 0.000000000000000000, 1.000000000000000000 ) ) ;
#36351=ORIENTED_EDGE ( 'NONE', *, *, #15952, .T. ) ;
#36450=CYLINDRICAL_SURFACE ( 'NONE', #40327, 4.999999999999997335 ) ;
#36665=AXIS2_PLACEMENT_3D ( 'NONE', #22203, #53501, #68989 ) ;
#36882=FILL_AREA_STYLE ('',( #15422 ) ) ;
#36952=EDGE_LOOP ( 'NONE', ( #48614, #58773, #29285, #63813 ) ) ;
#37027=DIRECTION ( 'NONE',  ( -0.000000000000000000, -0.000000000000000000, -1.000000000000000000 ) ) ;
#37043=CARTESIAN_POINT ( 'NONE',  ( 32.68347998332510684, -12.52158680757303344, 30.00000000000000000 ) ) ;
#37063=DIRECTION ( 'NONE',  ( -0.000000000000000000, 0.000000000000000000, -1.000000000000000000 ) ) ;
#37116=CYLINDRICAL_SURFACE ( 'NONE', #20997, 35.00000000000000000 ) ;
#37209=PRESENTATION_STYLE_ASSIGNMENT (( #15762 ) ) ;
#37244=DIRECTION ( 'NONE',  ( -0.000000000000000000, -0.000000000000000000, -1.000000000000000000 ) ) ;
#37579=ORIENTED_EDGE ( 'NONE', *, *, #42065, .T. ) ;
#37601=ORIENTED_EDGE ( 'NONE', *, *, #17794, .F. ) ;
#37619=EDGE_CURVE ( 'NONE', #47435, #8388, #794, .T. ) ;
#37921=DIRECTION ( 'NONE',  ( 0.000000000000000000, 1.000000000000000000, -0.000000000000000000 ) ) ;
#37942=DIRECTION ( 'NONE',  ( -1.000000000000000000, 0.000000000000000000, 0.000000000000000000 ) ) ;
#37968=CARTESIAN_POINT ( 'NONE',  ( 32.02161712141799654, -16.09918303830818687, 30.00000000000000000 ) ) ;
#37988=DIRECTION ( 'NONE',  ( -0.000000000000000000, 1.000000000000000000, -0.000000000000000000 ) ) ;
#38005=CARTESIAN_POINT ( 'NONE',  ( -25.00000000000000000, 0.000000000000000000, 30.00000000000000000 ) ) ;
#38171=CARTESIAN_POINT ( 'NONE',  ( 32.02161712141799654, -16.09918303830818687, 30.00000000000000000 ) ) ;
#38277=CARTESIAN_POINT ( 'NONE',  ( 0.000000000000000000, 0.000000000000000000, 30.00000000000000000 ) ) ;
#38287=CARTESIAN_POINT ( 'NONE',  ( 0.000000000000000000, 0.000000000000000000, 30.00000000000000000 ) ) ;
#38324=AXIS2_PLACEMENT_3D ( 'NONE', #44041, #65886, #39475 ) ;
#38404=ORIENTED_EDGE ( 'NONE', *, *, #63637, .T. ) ;
#38471=VERTEX_POINT ( 'NONE', #18201 ) ;
#38484=AXIS2_PLACEMENT_3D ( 'NONE', #21026, #26980, #69201 ) ;
#38523=CIRCLE ( 'NONE', #8209, 4.999999999999997335 ) ;
#38579=ORIENTED_EDGE ( 'NONE', *, *, #11924, .F. ) ;
#38724=DIRECTION ( 'NONE',  ( 0.000000000000000000, -0.000000000000000000, 1.000000000000000000 ) ) ;
#38788=ORIENTED_EDGE ( 'NONE', *, *, #30254, .F. ) ;
#38830=ADVANCED_FACE ( 'NONE', ( #55654, #50032 ), #55302, .T. ) ;
#38892=PRODUCT_DEFINITION_FORMATION_WITH_SPECIFIED_SOURCE ( 'ANY', '', #43365, .NOT_KNOWN. ) ;
#38914=DIRECTION ( 'NONE',  ( -0.000000000000000000, -0.000000000000000000, -1.000000000000000000 ) ) ;
#39433=DIRECTION ( 'NONE',  ( -0.000000000000000000, 1.000000000000000000, -0.000000000000000000 ) ) ;
#39475=DIRECTION ( 'NONE',  ( 1.000000000000000000, 0.000000000000000000, 0.000000000000000000 ) ) ;
#39572=DIRECTION ( 'NONE',  ( -0.000000000000000000, 0.000000000000000000, 1.000000000000000000 ) ) ;
#39679=ORIENTED_EDGE ( 'NONE', *, *, #32224, .F. ) ;
#39684=EDGE_CURVE ( 'NONE', #38471, #69231, #11646, .T. ) ;
#39688=DIRECTION ( 'NONE',  ( 1.000000000000000000, 0.000000000000000000, 0.000000000000000000 ) ) ;
#39776=EDGE_CURVE ( 'NONE', #19186, #69231, #38523, .T. ) ;
#39787=LINE ( 'NONE', #56658, #5793 ) ;
#39862=ORIENTED_EDGE ( 'NONE', *, *, #69144, .F. ) ;
#40117=CARTESIAN_POINT ( 'NONE',  ( -49.42000000000000171, -36.09918303830819752, 10.41169613715280740 ) ) ;
#40238=CIRCLE ( 'NONE', #52580, 35.00000000000000000 ) ;
#40327=AXIS2_PLACEMENT_3D ( 'NONE', #20961, #42412, #25902 ) ;
#40490=AXIS2_PLACEMENT_3D ( 'NONE', #28081, #49524, #61146 ) ;
#40574=DIRECTION ( 'NONE',  ( 0.000000000000000000, -1.000000000000000000, 0.000000000000000000 ) ) ;
#40688=VERTEX_POINT ( 'NONE', #51820 ) ;
#40710=ORIENTED_EDGE ( 'NONE', *, *, #7470, .T. ) ;
#40837=CARTESIAN_POINT ( 'NONE',  ( 68.07999999999999829, 0.000000000000000000, 0.000000000000000000 ) ) ;
#40951=VECTOR ( 'NONE', #44500, 1000.000000000000000 ) ;
#41087=ORIENTED_EDGE ( 'NONE', *, *, #5937, .T. ) ;
#41226=CARTESIAN_POINT ( 'NONE',  ( -32.68347998332510684, -12.52158680757305298, 0.000000000000000000 ) ) ;
#41377=SHAPE_DEFINITION_REPRESENTATION ( #15268, #52783 ) ;
#41479=CYLINDRICAL_SURFACE ( 'NONE', #55501, 4.999999999999997335 ) ;
#41589=ORIENTED_EDGE ( 'NONE', *, *, #30254, .T. ) ;
#41734=CARTESIAN_POINT ( 'NONE',  ( 42.02161712141799654, -16.09918303830818687, 30.00000000000000000 ) ) ;
#42065=EDGE_CURVE ( 'NONE', #2060, #64129, #27355, .T. ) ;
#42155=VERTEX_POINT ( 'NONE', #59107 ) ;
#42188=EDGE_CURVE ( 'NONE', #68800, #40688, #23241, .T. ) ;
#42344=FACE_OUTER_BOUND ( 'NONE', #62139, .T. ) ;
#42412=DIRECTION ( 'NONE',  ( -0.000000000000000000, 1.000000000000000000, -0.000000000000000000 ) ) ;
#42435=ORIENTED_EDGE ( 'NONE', *, *, #47943, .F. ) ;
#42718=EDGE_CURVE ( 'NONE', #27634, #59026, #65643, .T. ) ;
#43365=PRODUCT ( 'bearing', 'bearing', '', ( #19921 ) ) ;
#43707=EDGE_CURVE ( 'NONE', #47435, #34582, #3274, .T. ) ;
#43766=ORIENTED_EDGE ( 'NONE', *, *, #33919, .T. ) ;
#43835=AXIS2_PLACEMENT_3D ( 'NONE', #33018, #43903, #39688 ) ;
#43876=EDGE_CURVE ( 'NONE', #42155, #49926, #33811, .T. ) ;
#43903=DIRECTION ( 'NONE',  ( -0.000000000000000000, 0.000000000000000000, 1.000000000000000000 ) ) ;
#43979=CARTESIAN_POINT ( 'NONE',  ( 0.000000000000000000, -26.09918303830819397, 30.00000000000000000 ) ) ;
#44041=CARTESIAN_POINT ( 'NONE',  ( 0.000000000000000000, 0.000000000000000000, 0.000000000000000000 ) ) ;
#44217=EDGE_LOOP ( 'NONE', ( #17421, #51575, #48143, #26469 ) ) ;
#44379=CARTESIAN_POINT ( 'NONE',  ( -49.42000000000000171, -26.09918303830819397, 15.41169613715280562 ) ) ;
#44500=DIRECTION ( 'NONE',  ( -0.000000000000000000, -0.000000000000000000, -1.000000000000000000 ) ) ;
#44558=DIRECTION ( 'NONE',  ( 0.000000000000000000, 0.000000000000000000, 1.000000000000000000 ) ) ;
#44606=DIRECTION ( 'NONE',  ( -1.000000000000000000, 0.000000000000000000, 0.000000000000000000 ) ) ;
#44649=VECTOR ( 'NONE', #4581, 1000.000000000000000 ) ;
#44838=ORIENTED_EDGE ( 'NONE', *, *, #16095, .F. ) ;
#44864=CARTESIAN_POINT ( 'NONE',  ( 0.000000000000000000, 0.000000000000000000, 30.00000000000000000 ) ) ;
#45328=CARTESIAN_POINT ( 'NONE',  ( 25.00000000000000000, 3.061616997868383043E-15, 30.00000000000000000 ) ) ;
#45354=ADVANCED_FACE ( 'NONE', ( #3268, #15197 ), #62351, .T. ) ;
#45777=LINE ( 'NONE', #40837, #63342 ) ;
#45835=ORIENTED_EDGE ( 'NONE', *, *, #45908, .T. ) ;
#45908=EDGE_CURVE ( 'NONE', #42155, #64838, #61495, .T. ) ;
#46101=CARTESIAN_POINT ( 'NONE',  ( -25.00000000000000000, 0.000000000000000000, 30.00000000000000000 ) ) ;
#46687=CARTESIAN_POINT ( 'NONE',  ( 68.07999999999999829, -36.09918303830819752, 30.00000000000000000 ) ) ;
#47330=CARTESIAN_POINT ( 'NONE',  ( 0.000000000000000000, -36.09918303830819752, 30.00000000000000000 ) ) ;
#47338=DIRECTION ( 'NONE',  ( -0.000000000000000000, 0.000000000000000000, -1.000000000000000000 ) ) ;
#47356=VECTOR ( 'NONE', #48161, 1000.000000000000000 ) ;
#47377=VERTEX_POINT ( 'NONE', #23630 ) ;
#47435=VERTEX_POINT ( 'NONE', #22576 ) ;
#47468=VECTOR ( 'NONE', #38914, 1000.000000000000000 ) ;
#47533=CARTESIAN_POINT ( 'NONE',  ( 42.02161712141799654, -26.09918303830819042, 30.00000000000000000 ) ) ;
#47618=EDGE_CURVE ( 'NONE', #8388, #10885, #55094, .T. ) ;
#47807=( GEOMETRIC_REPRESENTATION_CONTEXT ( 3 ) GLOBAL_UNCERTAINTY_ASSIGNED_CONTEXT ( ( #4337 ) ) GLOBAL_UNIT_ASSIGNED_CONTEXT ( ( #21203, #80, #64450 ) ) REPRESENTATION_CONTEXT ( 'NONE', 'WORKASPACE' ) );
#47865=ORIENTED_EDGE ( 'NONE', *, *, #33555, .T. ) ;
#47943=EDGE_CURVE ( 'NONE', #40688, #11023, #67210, .T. ) ;
#47951=CARTESIAN_POINT ( 'NONE',  ( 32.68347998332510684, -12.52158680757303344, 30.00000000000000000 ) ) ;
#48143=ORIENTED_EDGE ( 'NONE', *, *, #18028, .T. ) ;
#48161=DIRECTION ( 'NONE',  ( 0.000000000000000000, -1.000000000000000000, 0.000000000000000000 ) ) ;
#48195=VECTOR ( 'NONE', #21159, 1000.000000000000000 ) ;
#48577=ORIENTED_EDGE ( 'NONE', *, *, #47618, .F. ) ;
#48580=CARTESIAN_POINT ( 'NONE',  ( 68.07999999999999829, -26.09918303830819397, 30.00000000000000000 ) ) ;
#48581=PRODUCT_DEFINITION_CONTEXT ( 'detailed design', #9390, 'design' ) ;
#48614=ORIENTED_EDGE ( 'NONE', *, *, #62427, .T. ) ;
#48733=ORIENTED_EDGE ( 'NONE', *, *, #2101, .T. ) ;
#48791=DIRECTION ( 'NONE',  ( 0.000000000000000000, 0.000000000000000000, 1.000000000000000000 ) ) ;
#48974=DIRECTION ( 'NONE',  ( 0.000000000000000000, 1.000000000000000000, -0.000000000000000000 ) ) ;
#49067=CARTESIAN_POINT ( 'NONE',  ( -42.02161712141799654, -16.09918303830819397, 30.00000000000000000 ) ) ;
#49318=EDGE_LOOP ( 'NONE', ( #15524, #62754, #62072, #45835 ) ) ;
#49324=ORIENTED_EDGE ( 'NONE', *, *, #62827, .T. ) ;
#49524=DIRECTION ( 'NONE',  ( 0.000000000000000000, -0.000000000000000000, -1.000000000000000000 ) ) ;
#49558=ORIENTED_EDGE ( 'NONE', *, *, #22731, .T. ) ;
#49631=CLOSED_SHELL ( 'NONE', ( #5137, #32235, #66203, #64019, #29620, #6804, #7385, #56547, #2389, #56731, #38830, #19322, #29556, #33207, #34294, #45354, #57023, #9565, #6359 ) ) ;
#49713=LINE ( 'NONE', #1543, #52057 ) ;
#49715=VERTEX_POINT ( 'NONE', #62221 ) ;
#49926=VERTEX_POINT ( 'NONE', #15428 ) ;
#49970=DIRECTION ( 'NONE',  ( -0.000000000000000000, 0.000000000000000000, 1.000000000000000000 ) ) ;
#49974=VECTOR ( 'NONE', #8044, 1000.000000000000000 ) ;
#50032=FACE_OUTER_BOUND ( 'NONE', #32160, .T. ) ;
#50255=ORIENTED_EDGE ( 'NONE', *, *, #54212, .T. ) ;
#50273=CARTESIAN_POINT ( 'NONE',  ( 0.000000000000000000, 0.000000000000000000, 30.00000000000000000 ) ) ;
#50281=VECTOR ( 'NONE', #40574, 1000.000000000000000 ) ;
#50353=FACE_BOUND ( 'NONE', #8554, .T. ) ;
#50472=DIRECTION ( 'NONE',  ( 1.000000000000000000, 0.000000000000000000, 0.000000000000000000 ) ) ;
#50530=CARTESIAN_POINT ( 'NONE',  ( 0.000000000000000000, 0.000000000000000000, 0.000000000000000000 ) ) ;
#50749=VECTOR ( 'NONE', #50996, 1000.000000000000000 ) ;
#50946=ORIENTED_EDGE ( 'NONE', *, *, #6019, .F. ) ;
#50996=DIRECTION ( 'NONE',  ( -0.000000000000000000, -0.000000000000000000, -1.000000000000000000 ) ) ;
#51430=VERTEX_POINT ( 'NONE', #28152 ) ;
#51575=ORIENTED_EDGE ( 'NONE', *, *, #42065, .F. ) ;
#51587=CARTESIAN_POINT ( 'NONE',  ( 0.000000000000000000, 0.000000000000000000, 0.000000000000000000 ) ) ;
#51589=STYLED_ITEM ( 'NONE', ( #37209 ), #64527 ) ;
#51757=DIRECTION ( 'NONE',  ( 1.000000000000000000, 0.000000000000000000, 0.000000000000000000 ) ) ;
#51763=ORIENTED_EDGE ( 'NONE', *, *, #47943, .T. ) ;
#51820=CARTESIAN_POINT ( 'NONE',  ( -25.00000000000000000, 0.000000000000000000, 0.000000000000000000 ) ) ;
#51859=CYLINDRICAL_SURFACE ( 'NONE', #24624, 25.00000000000000000 ) ;
#52057=VECTOR ( 'NONE', #65938, 1000.000000000000000 ) ;
#52373=DIRECTION ( 'NONE',  ( 1.000000000000000000, 0.000000000000000000, 0.000000000000000000 ) ) ;
#52380=DIRECTION ( 'NONE',  ( -0.000000000000000000, 0.000000000000000000, 1.000000000000000000 ) ) ;
#52580=AXIS2_PLACEMENT_3D ( 'NONE', #64150, #10336, #32148 ) ;
#52624=FACE_OUTER_BOUND ( 'NONE', #9517, .T. ) ;
#52625=CARTESIAN_POINT ( 'NONE',  ( -56.92000000000000171, 0.000000000000000000, 30.00000000000000000 ) ) ;
#52695=EDGE_LOOP ( 'NONE', ( #8596, #28818, #39679, #47865 ) ) ;
#52783=SHAPE_REPRESENTATION ( 'bearing', ( #66832 ), #47807 ) ;
#52968=FACE_OUTER_BOUND ( 'NONE', #8085, .T. ) ;
#53201=DIRECTION ( 'NONE',  ( 0.000000000000000000, 0.000000000000000000, 1.000000000000000000 ) ) ;
#53254=EDGE_CURVE ( 'NONE', #68965, #47435, #63254, .T. ) ;
#53436=LINE ( 'NONE', #5265, #49974 ) ;
#53448=DIRECTION ( 'NONE',  ( 1.000000000000000000, 0.000000000000000000, 0.000000000000000000 ) ) ;
#53501=DIRECTION ( 'NONE',  ( -0.000000000000000000, 0.000000000000000000, 1.000000000000000000 ) ) ;
#53574=CARTESIAN_POINT ( 'NONE',  ( -56.92000000000000171, -36.09918303830819752, 30.00000000000000000 ) ) ;
#53883=EDGE_CURVE ( 'NONE', #60359, #56353, #54273, .T. ) ;
#54010=DIRECTION ( 'NONE',  ( 0.000000000000000000, 1.000000000000000000, -0.000000000000000000 ) ) ;
#54147=CARTESIAN_POINT ( 'NONE',  ( 35.00000000000000000, 4.286263797015736496E-15, 0.000000000000000000 ) ) ;
#54212=EDGE_CURVE ( 'NONE', #64129, #2060, #62134, .T. ) ;
#54248=CARTESIAN_POINT ( 'NONE',  ( -49.42000000000000171, -36.09918303830819752, 15.41169613715280562 ) ) ;
#54273=CIRCLE ( 'NONE', #55399, 4.999999999999997335 ) ;
#54347=DIRECTION ( 'NONE',  ( -0.000000000000000000, -0.000000000000000000, -1.000000000000000000 ) ) ;
#54403=CARTESIAN_POINT ( 'NONE',  ( -49.42000000000000171, -36.09918303830819752, 15.41169613715280562 ) ) ;
#54702=CYLINDRICAL_SURFACE ( 'NONE', #5519, 9.999999999999994671 ) ;
#54729=AXIS2_PLACEMENT_3D ( 'NONE', #32991, #65716, #33357 ) ;
#54757=DIRECTION ( 'NONE',  ( 0.000000000000000000, 1.000000000000000000, -0.000000000000000000 ) ) ;
#54796=VERTEX_POINT ( 'NONE', #37043 ) ;
#54958=DIRECTION ( 'NONE',  ( 0.000000000000000000, 0.000000000000000000, 1.000000000000000000 ) ) ;
#55000=EDGE_CURVE ( 'NONE', #62166, #34582, #67821, .T. ) ;
#55094=LINE ( 'NONE', #66035, #44649 ) ;
#55096=DIRECTION ( 'NONE',  ( -0.000000000000000000, -0.000000000000000000, -1.000000000000000000 ) ) ;
#55152=AXIS2_PLACEMENT_3D ( 'NONE', #1272, #54010, #5839 ) ;
#55170=VERTEX_POINT ( 'NONE', #54147 ) ;
#55302=PLANE ( 'NONE',  #34018 ) ;
#55399=AXIS2_PLACEMENT_3D ( 'NONE', #44379, #17301, #27157 ) ;
#55501=AXIS2_PLACEMENT_3D ( 'NONE', #14404, #62226, #23912 ) ;
#55654=FACE_BOUND ( 'NONE', #3390, .T. ) ;
#56100=CARTESIAN_POINT ( 'NONE',  ( 42.02161712141799654, -16.09918303830818687, 30.00000000000000000 ) ) ;
#56258=FACE_OUTER_BOUND ( 'NONE', #67126, .T. ) ;
#56338=CARTESIAN_POINT ( 'NONE',  ( 42.02161712141799654, -16.09918303830818687, 0.000000000000000000 ) ) ;
#56353=VERTEX_POINT ( 'NONE', #30843 ) ;
#56547=ADVANCED_FACE ( 'NONE', ( #5478 ), #31193, .F. ) ;
#56654=DIRECTION ( 'NONE',  ( 0.000000000000000000, 1.000000000000000000, -0.000000000000000000 ) ) ;
#56658=CARTESIAN_POINT ( 'NONE',  ( 0.000000000000000000, -36.09918303830819752, 0.000000000000000000 ) ) ;
#56667=ORIENTED_EDGE ( 'NONE', *, *, #42718, .T. ) ;
#56674=DIRECTION ( 'NONE',  ( 0.000000000000000000, -1.000000000000000000, 0.000000000000000000 ) ) ;
#56731=ADVANCED_FACE ( 'NONE', ( #42344 ), #4023, .T. ) ;
#56777=VERTEX_POINT ( 'NONE', #5047 ) ;
#56858=CARTESIAN_POINT ( 'NONE',  ( -35.00000000000000000, 0.000000000000000000, 0.000000000000000000 ) ) ;
#57023=ADVANCED_FACE ( 'NONE', ( #25318, #20033 ), #58005, .F. ) ;
#57315=DIRECTION ( 'NONE',  ( 1.000000000000000000, 0.000000000000000000, 0.000000000000000000 ) ) ;
#57333=DIRECTION ( 'NONE',  ( -0.000000000000000000, 1.000000000000000000, -0.000000000000000000 ) ) ;
#57571=CYLINDRICAL_SURFACE ( 'NONE', #21493, 10.00000000000000178 ) ;
#57730=AXIS2_PLACEMENT_3D ( 'NONE', #8134, #62286, #66896 ) ;
#57834=DIRECTION ( 'NONE',  ( 1.000000000000000000, 0.000000000000000000, -0.000000000000000000 ) ) ;
#57870=AXIS2_PLACEMENT_3D ( 'NONE', #3166, #52380, #57315 ) ;
#57872=AXIS2_PLACEMENT_3D ( 'NONE', #4795, #54347, #27276 ) ;
#58005=PLANE ( 'NONE',  #57870 ) ;
#58084=ORIENTED_EDGE ( 'NONE', *, *, #94, .T. ) ;
#58107=VECTOR ( 'NONE', #19717, 1000.000000000000000 ) ;
#58157=CARTESIAN_POINT ( 'NONE',  ( -49.42000000000000171, -26.09918303830819397, 15.41169613715280562 ) ) ;
#58507=LINE ( 'NONE', #53574, #14569 ) ;
#58773=ORIENTED_EDGE ( 'NONE', *, *, #33919, .F. ) ;
#58971=EDGE_LOOP ( 'NONE', ( #51763, #22765 ) ) ;
#59026=VERTEX_POINT ( 'NONE', #66960 ) ;
#59107=CARTESIAN_POINT ( 'NONE',  ( -56.92000000000000171, -26.09918303830819397, 30.00000000000000000 ) ) ;
#59518=DIRECTION ( 'NONE',  ( 0.000000000000000000, 1.000000000000000000, -0.000000000000000000 ) ) ;
#59558=EDGE_LOOP ( 'NONE', ( #44838, #2467, #14703, #6014 ) ) ;
#59646=CARTESIAN_POINT ( 'NONE',  ( 25.00000000000000000, 3.061616997868383043E-15, 0.000000000000000000 ) ) ;
#59649=CIRCLE ( 'NONE', #38324, 35.00000000000000000 ) ;
#59706=VECTOR ( 'NONE', #37988, 1000.000000000000000 ) ;
#59722=FACE_OUTER_BOUND ( 'NONE', #61555, .T. ) ;
#59838=ORIENTED_EDGE ( 'NONE', *, *, #43707, .F. ) ;
#60171=VERTEX_POINT ( 'NONE', #56858 ) ;
#60200=EDGE_LOOP ( 'NONE', ( #62645, #842 ) ) ;
#60252=VECTOR ( 'NONE', #29477, 1000.000000000000000 ) ;
#60359=VERTEX_POINT ( 'NONE', #11066 ) ;
#60396=LINE ( 'NONE', #7284, #9217 ) ;
#60545=CARTESIAN_POINT ( 'NONE',  ( 35.00000000000000000, 4.286263797015736496E-15, 30.00000000000000000 ) ) ;
#61011=CARTESIAN_POINT ( 'NONE',  ( 68.07999999999999829, -26.09918303830819397, 0.000000000000000000 ) ) ;
#61069=ORIENTED_EDGE ( 'NONE', *, *, #32224, .T. ) ;
#61146=DIRECTION ( 'NONE',  ( 1.000000000000000000, 0.000000000000000000, 0.000000000000000000 ) ) ;
#61208=DIRECTION ( 'NONE',  ( -0.000000000000000000, 1.000000000000000000, -0.000000000000000000 ) ) ;
#61244=CARTESIAN_POINT ( 'NONE',  ( 60.58000000000000540, -26.09918303830819397, 15.41169613715280562 ) ) ;
#61287=AXIS2_PLACEMENT_3D ( 'NONE', #43979, #17253, #38724 ) ;
#61481=ORIENTED_EDGE ( 'NONE', *, *, #22731, .F. ) ;
#61495=LINE ( 'NONE', #13645, #60252 ) ;
#61547=EDGE_CURVE ( 'NONE', #56353, #60359, #69297, .T. ) ;
#61552=CYLINDRICAL_SURFACE ( 'NONE', #4990, 4.999999999999997335 ) ;
#61555=EDGE_LOOP ( 'NONE', ( #38579, #36351, #3419, #24378 ) ) ;
#61671=MECHANICAL_DESIGN_GEOMETRIC_PRESENTATION_REPRESENTATION('',(#51589),#10006);
#61686=DIRECTION ( 'NONE',  ( -0.000000000000000000, 0.000000000000000000, 1.000000000000000000 ) ) ;
#61861=ORIENTED_EDGE ( 'NONE', *, *, #5937, .F. ) ;
#61890=CARTESIAN_POINT ( 'NONE',  ( 60.58000000000000540, -36.09918303830819752, 10.41169613715280740 ) ) ;
#61901=LINE ( 'NONE', #40117, #27578 ) ;
#62072=ORIENTED_EDGE ( 'NONE', *, *, #30171, .F. ) ;
#62134=CIRCLE ( 'NONE', #26184, 4.999999999999997335 ) ;
#62139=EDGE_LOOP ( 'NONE', ( #17493, #61481, #5120, #58084 ) ) ;
#62145=DIRECTION ( 'NONE',  ( -1.000000000000000000, 0.000000000000000000, 0.000000000000000000 ) ) ;
#62166=VERTEX_POINT ( 'NONE', #35692 ) ;
#62221=CARTESIAN_POINT ( 'NONE',  ( 68.07999999999999829, -36.09918303830819752, 0.000000000000000000 ) ) ;
#62226=DIRECTION ( 'NONE',  ( -0.000000000000000000, 1.000000000000000000, -0.000000000000000000 ) ) ;
#62286=DIRECTION ( 'NONE',  ( 0.000000000000000000, 1.000000000000000000, 0.000000000000000000 ) ) ;
#62351=PLANE ( 'NONE',  #36665 ) ;
#62427=EDGE_CURVE ( 'NONE', #66426, #47377, #4189, .T. ) ;
#62645=ORIENTED_EDGE ( 'NONE', *, *, #53883, .F. ) ;
#62754=ORIENTED_EDGE ( 'NONE', *, *, #33555, .F. ) ;
#62827=EDGE_CURVE ( 'NONE', #54796, #56777, #25837, .T. ) ;
#62917=EDGE_CURVE ( 'NONE', #60171, #66426, #34585, .T. ) ;
#63049=ORIENTED_EDGE ( 'NONE', *, *, #66746, .F. ) ;
#63254=CIRCLE ( 'NONE', #38484, 10.00000000000000178 ) ;
#63342=VECTOR ( 'NONE', #56674, 1000.000000000000000 ) ;
#63383=ORIENTED_EDGE ( 'NONE', *, *, #16636, .F. ) ;
#63460=DIRECTION ( 'NONE',  ( -0.000000000000000000, -0.000000000000000000, -1.000000000000000000 ) ) ;
#63509=CARTESIAN_POINT ( 'NONE',  ( 0.000000000000000000, 0.000000000000000000, 30.00000000000000000 ) ) ;
#63637=EDGE_CURVE ( 'NONE', #59026, #69403, #40238, .T. ) ;
#63710=EDGE_LOOP ( 'NONE', ( #63049, #38788, #2987, #63930 ) ) ;
#63713=ORIENTED_EDGE ( 'NONE', *, *, #43876, .F. ) ;
#63813=ORIENTED_EDGE ( 'NONE', *, *, #69144, .T. ) ;
#63890=ORIENTED_EDGE ( 'NONE', *, *, #53254, .F. ) ;
#63930=ORIENTED_EDGE ( 'NONE', *, *, #321, .T. ) ;
#64019=ADVANCED_FACE ( 'NONE', ( #27731 ), #11201, .T. ) ;
#64129=VERTEX_POINT ( 'NONE', #17887 ) ;
#64135=CARTESIAN_POINT ( 'NONE',  ( 68.07999999999999829, 0.000000000000000000, 30.00000000000000000 ) ) ;
#64150=CARTESIAN_POINT ( 'NONE',  ( 0.000000000000000000, 0.000000000000000000, 30.00000000000000000 ) ) ;
#64206=LINE ( 'NONE', #47330, #66160 ) ;
#64244=ORIENTED_EDGE ( 'NONE', *, *, #30518, .F. ) ;
#64450=( NAMED_UNIT ( * ) SI_UNIT ( $, .STERADIAN. ) SOLID_ANGLE_UNIT ( ) );
#64527=MANIFOLD_SOLID_BREP ( 'Cut-Extrude1', #49631 ) ;
#64796=LINE ( 'NONE', #48580, #22917 ) ;
#64838=VERTEX_POINT ( 'NONE', #16364 ) ;
#65328=ORIENTED_EDGE ( 'NONE', *, *, #42718, .F. ) ;
#65373=DIRECTION ( 'NONE',  ( -0.000000000000000000, -0.000000000000000000, -1.000000000000000000 ) ) ;
#65426=ORIENTED_EDGE ( 'NONE', *, *, #53254, .T. ) ;
#65643=CIRCLE ( 'NONE', #20692, 35.00000000000000000 ) ;
#65675=LINE ( 'NONE', #23802, #16225 ) ;
#65716=DIRECTION ( 'NONE',  ( 0.000000000000000000, -0.000000000000000000, -1.000000000000000000 ) ) ;
#65725=DIRECTION ( 'NONE',  ( 0.000000000000000000, 0.000000000000000000, 1.000000000000000000 ) ) ;
#65886=DIRECTION ( 'NONE',  ( -0.000000000000000000, 0.000000000000000000, 1.000000000000000000 ) ) ;
#65938=DIRECTION ( 'NONE',  ( 1.000000000000000000, 0.000000000000000000, 0.000000000000000000 ) ) ;
#65951=DIRECTION ( 'NONE',  ( 1.000000000000000000, 0.000000000000000000, 0.000000000000000000 ) ) ;
#66035=CARTESIAN_POINT ( 'NONE',  ( 68.07999999999999829, 0.000000000000000000, 30.00000000000000000 ) ) ;
#66037=ORIENTED_EDGE ( 'NONE', *, *, #22963, .T. ) ;
#66160=VECTOR ( 'NONE', #68788, 1000.000000000000000 ) ;
#66203=ADVANCED_FACE ( 'NONE', ( #8957 ), #51859, .F. ) ;
#66238=DIRECTION ( 'NONE',  ( 0.000000000000000000, 1.000000000000000000, 0.000000000000000000 ) ) ;
#66254=DIRECTION ( 'NONE',  ( 1.000000000000000000, 0.000000000000000000, 0.000000000000000000 ) ) ;
#66334=CIRCLE ( 'NONE', #43835, 10.00000000000000178 ) ;
#66426=VERTEX_POINT ( 'NONE', #41226 ) ;
#66746=EDGE_CURVE ( 'NONE', #51430, #19186, #24280, .T. ) ;
#66832=AXIS2_PLACEMENT_3D ( 'NONE', #50530, #44558, #8319 ) ;
#66868=ORIENTED_EDGE ( 'NONE', *, *, #19067, .F. ) ;
#66896=DIRECTION ( 'NONE',  ( 0.000000000000000000, -0.000000000000000000, 1.000000000000000000 ) ) ;
#66960=CARTESIAN_POINT ( 'NONE',  ( -35.00000000000000000, 0.000000000000000000, 30.00000000000000000 ) ) ;
#67038=DIRECTION ( 'NONE',  ( -0.000000000000000000, 0.000000000000000000, 1.000000000000000000 ) ) ;
#67126=EDGE_LOOP ( 'NONE', ( #26697, #40710, #18308, #14738 ) ) ;
#67161=CARTESIAN_POINT ( 'NONE',  ( 60.58000000000000540, -26.09918303830819397, 20.41169613715280207 ) ) ;
#67210=CIRCLE ( 'NONE', #15522, 25.00000000000000000 ) ;
#67361=DIRECTION ( 'NONE',  ( 1.000000000000000000, 0.000000000000000000, 0.000000000000000000 ) ) ;
#67378=ORIENTED_EDGE ( 'NONE', *, *, #321, .F. ) ;
#67821=CIRCLE ( 'NONE', #3791, 10.00000000000000178 ) ;
#67920=LINE ( 'NONE', #35554, #58107 ) ;
#68016=LINE ( 'NONE', #35999, #50281 ) ;
#68260=APPLICATION_CONTEXT ( 'automotive_design' ) ;
#68788=DIRECTION ( 'NONE',  ( 1.000000000000000000, 0.000000000000000000, 0.000000000000000000 ) ) ;
#68800=VERTEX_POINT ( 'NONE', #46101 ) ;
#68965=VERTEX_POINT ( 'NONE', #37968 ) ;
#68989=DIRECTION ( 'NONE',  ( 1.000000000000000000, 0.000000000000000000, 0.000000000000000000 ) ) ;
#69064=ORIENTED_EDGE ( 'NONE', *, *, #55000, .F. ) ;
#69144=EDGE_CURVE ( 'NONE', #69403, #66426, #53436, .T. ) ;
#69201=DIRECTION ( 'NONE',  ( 1.000000000000000000, 0.000000000000000000, 0.000000000000000000 ) ) ;
#69210=VERTEX_POINT ( 'NONE', #45328 ) ;
#69231=VERTEX_POINT ( 'NONE', #67161 ) ;
#69297=CIRCLE ( 'NONE', #23230, 4.999999999999997335 ) ;
#69336=LINE ( 'NONE', #20804, #48195 ) ;
#69400=ORIENTED_EDGE ( 'NONE', *, *, #901, .T. ) ;
#69403=VERTEX_POINT ( 'NONE', #5525 ) ;
#69569=EDGE_CURVE ( 'NONE', #27634, #55170, #65675, .T. ) ;
ENDSEC;
END-ISO-10303-21;
